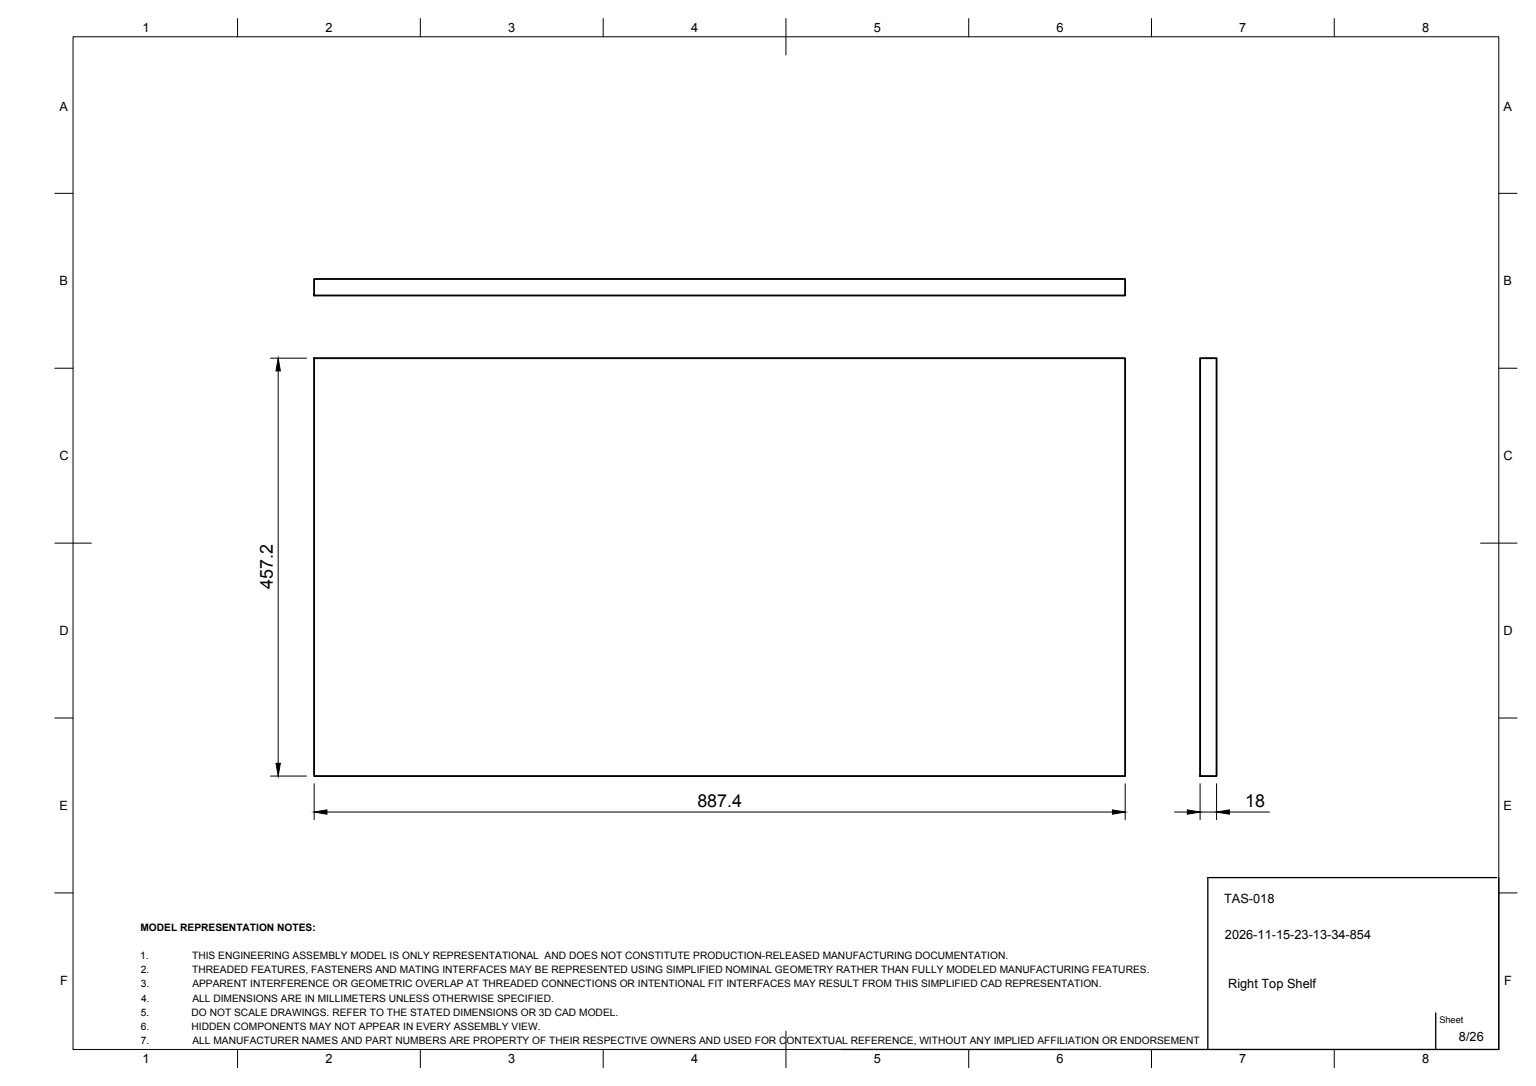
ISO-10303-21;
HEADER;
/* Generated by software containing ST-Developer
 * from STEP Tools, Inc. (www.steptools.com) 
 */

FILE_DESCRIPTION(
/* description */ (''),
/* implementation_level */ '2;1');

FILE_NAME(
/* name */ 'Right Top Shelf.step',
/* time_stamp */ '2026-11-15T15:17:57-08:00',
/* author */ (''),
/* organization */ (''),
/* preprocessor_version */ 'ST-DEVELOPER v20.2',
/* originating_system */ 'Autodesk Translation Framework v15.17.0.0',
/* authorisation */ '');

FILE_SCHEMA (('AUTOMOTIVE_DESIGN { 1 0 10303 214 3 1 1 }'));
ENDSEC;

DATA;
#10=MECHANICAL_DESIGN_GEOMETRIC_PRESENTATION_REPRESENTATION('',(#183),#3723);
#135=SHAPE_REPRESENTATION_RELATIONSHIP('SRR','None',#3816,#159);
#159=ADVANCED_BREP_SHAPE_REPRESENTATION('',(#207),#3705);
#183=STYLED_ITEM('',(#3947),#207);
#207=MANIFOLD_SOLID_BREP('Body1',#2031);
#258=FACE_OUTER_BOUND('',#384,.T.);
#259=FACE_OUTER_BOUND('',#385,.T.);
#260=FACE_OUTER_BOUND('',#386,.T.);
#261=FACE_OUTER_BOUND('',#387,.T.);
#262=FACE_OUTER_BOUND('',#388,.T.);
#263=FACE_OUTER_BOUND('',#389,.T.);
#384=EDGE_LOOP('',(#1437,#1438,#1439,#1440));
#385=EDGE_LOOP('',(#1441,#1442,#1443,#1444));
#386=EDGE_LOOP('',(#1445,#1446,#1447,#1448));
#387=EDGE_LOOP('',(#1449,#1450,#1451,#1452));
#388=EDGE_LOOP('',(#1453,#1454,#1455,#1456));
#389=EDGE_LOOP('',(#1457,#1458,#1459,#1460));
#538=LINE('',#3254,#760);
#539=LINE('',#3256,#761);
#540=LINE('',#3258,#762);
#541=LINE('',#3259,#763);
#542=LINE('',#3262,#764);
#543=LINE('',#3264,#765);
#544=LINE('',#3265,#766);
#545=LINE('',#3268,#767);
#546=LINE('',#3270,#768);
#547=LINE('',#3271,#769);
#548=LINE('',#3273,#770);
#549=LINE('',#3274,#771);
#760=VECTOR('',#2656,0.708661417322839);
#761=VECTOR('',#2657,18.);
#762=VECTOR('',#2658,0.708661417322839);
#763=VECTOR('',#2659,18.);
#764=VECTOR('',#2662,34.9370078740157);
#765=VECTOR('',#2663,18.);
#766=VECTOR('',#2664,34.9370078740157);
#767=VECTOR('',#2667,0.708661417322839);
#768=VECTOR('',#2668,18.);
#769=VECTOR('',#2669,0.708661417322839);
#770=VECTOR('',#2672,34.9370078740157);
#771=VECTOR('',#2673,34.9370078740157);
#963=VERTEX_POINT('',#3252);
#964=VERTEX_POINT('',#3253);
#965=VERTEX_POINT('',#3255);
#966=VERTEX_POINT('',#3257);
#967=VERTEX_POINT('',#3261);
#968=VERTEX_POINT('',#3263);
#969=VERTEX_POINT('',#3267);
#970=VERTEX_POINT('',#3269);
#1140=EDGE_CURVE('',#963,#964,#538,.T.);
#1141=EDGE_CURVE('',#965,#963,#539,.T.);
#1142=EDGE_CURVE('',#965,#966,#540,.T.);
#1143=EDGE_CURVE('',#966,#964,#541,.T.);
#1144=EDGE_CURVE('',#967,#963,#542,.T.);
#1145=EDGE_CURVE('',#968,#967,#543,.T.);
#1146=EDGE_CURVE('',#968,#965,#544,.T.);
#1147=EDGE_CURVE('',#967,#969,#545,.T.);
#1148=EDGE_CURVE('',#970,#969,#546,.T.);
#1149=EDGE_CURVE('',#968,#970,#547,.T.);
#1150=EDGE_CURVE('',#969,#964,#548,.T.);
#1151=EDGE_CURVE('',#970,#966,#549,.T.);
#1437=ORIENTED_EDGE('',*,*,#1140,.F.);
#1438=ORIENTED_EDGE('',*,*,#1141,.F.);
#1439=ORIENTED_EDGE('',*,*,#1142,.T.);
#1440=ORIENTED_EDGE('',*,*,#1143,.T.);
#1441=ORIENTED_EDGE('',*,*,#1144,.F.);
#1442=ORIENTED_EDGE('',*,*,#1145,.F.);
#1443=ORIENTED_EDGE('',*,*,#1146,.T.);
#1444=ORIENTED_EDGE('',*,*,#1141,.T.);
#1445=ORIENTED_EDGE('',*,*,#1147,.T.);
#1446=ORIENTED_EDGE('',*,*,#1148,.F.);
#1447=ORIENTED_EDGE('',*,*,#1149,.F.);
#1448=ORIENTED_EDGE('',*,*,#1145,.T.);
#1449=ORIENTED_EDGE('',*,*,#1150,.T.);
#1450=ORIENTED_EDGE('',*,*,#1143,.F.);
#1451=ORIENTED_EDGE('',*,*,#1151,.F.);
#1452=ORIENTED_EDGE('',*,*,#1148,.T.);
#1453=ORIENTED_EDGE('',*,*,#1142,.F.);
#1454=ORIENTED_EDGE('',*,*,#1146,.F.);
#1455=ORIENTED_EDGE('',*,*,#1149,.T.);
#1456=ORIENTED_EDGE('',*,*,#1151,.T.);
#1457=ORIENTED_EDGE('',*,*,#1140,.T.);
#1458=ORIENTED_EDGE('',*,*,#1150,.F.);
#1459=ORIENTED_EDGE('',*,*,#1147,.F.);
#1460=ORIENTED_EDGE('',*,*,#1144,.T.);
#1811=PLANE('',#2359);
#1812=PLANE('',#2360);
#1813=PLANE('',#2361);
#1814=PLANE('',#2362);
#1815=PLANE('',#2363);
#1816=PLANE('',#2364);
#1932=ADVANCED_FACE('',(#258),#1811,.T.);
#1933=ADVANCED_FACE('',(#259),#1812,.T.);
#1934=ADVANCED_FACE('',(#260),#1813,.F.);
#1935=ADVANCED_FACE('',(#261),#1814,.F.);
#1936=ADVANCED_FACE('',(#262),#1815,.T.);
#1937=ADVANCED_FACE('',(#263),#1816,.F.);
#2031=CLOSED_SHELL('',(#1932,#1933,#1934,#1935,#1936,#1937));
#2358=AXIS2_PLACEMENT_3D('',#3250,#2652,#2653);
#2359=AXIS2_PLACEMENT_3D('',#3251,#2654,#2655);
#2360=AXIS2_PLACEMENT_3D('',#3260,#2660,#2661);
#2361=AXIS2_PLACEMENT_3D('',#3266,#2665,#2666);
#2362=AXIS2_PLACEMENT_3D('',#3272,#2670,#2671);
#2363=AXIS2_PLACEMENT_3D('',#3275,#2674,#2675);
#2364=AXIS2_PLACEMENT_3D('',#3276,#2676,#2677);
#2652=DIRECTION('axis',(0.,0.,1.));
#2653=DIRECTION('refdir',(1.,0.,0.));
#2654=DIRECTION('center_axis',(1.,0.,0.));
#2655=DIRECTION('ref_axis',(0.,0.,-1.));
#2656=DIRECTION('',(0.,-1.,0.));
#2657=DIRECTION('',(0.,0.,-1.));
#2658=DIRECTION('',(0.,-1.,0.));
#2659=DIRECTION('',(0.,0.,-1.));
#2660=DIRECTION('center_axis',(0.,1.,0.));
#2661=DIRECTION('ref_axis',(0.,0.,1.));
#2662=DIRECTION('',(1.,0.,0.));
#2663=DIRECTION('',(0.,0.,-1.));
#2664=DIRECTION('',(1.,0.,0.));
#2665=DIRECTION('center_axis',(1.,0.,0.));
#2666=DIRECTION('ref_axis',(0.,0.,-1.));
#2667=DIRECTION('',(0.,-1.,0.));
#2668=DIRECTION('',(0.,0.,-1.));
#2669=DIRECTION('',(0.,-1.,0.));
#2670=DIRECTION('center_axis',(0.,1.,0.));
#2671=DIRECTION('ref_axis',(0.,0.,1.));
#2672=DIRECTION('',(1.,0.,0.));
#2673=DIRECTION('',(1.,0.,0.));
#2674=DIRECTION('center_axis',(0.,0.,1.));
#2675=DIRECTION('ref_axis',(1.,0.,0.));
#2676=DIRECTION('center_axis',(0.,0.,1.));
#2677=DIRECTION('ref_axis',(1.,0.,0.));
#3250=CARTESIAN_POINT('',(0.,0.,0.));
#3251=CARTESIAN_POINT('Origin',(35.2913385826772,0.,18.7086614173228));
#3252=CARTESIAN_POINT('',(35.2913385826772,67.3543307086614,0.708661417322834));
#3253=CARTESIAN_POINT('',(35.2913385826772,66.6456692913386,0.708661417322834));
#3254=CARTESIAN_POINT('',(35.2913385826772,67.3543307086614,0.708661417322834));
#3255=CARTESIAN_POINT('',(35.2913385826772,67.3543307086614,18.7086614173228));
#3256=CARTESIAN_POINT('',(35.2913385826772,67.3543307086614,18.7086614173228));
#3257=CARTESIAN_POINT('',(35.2913385826772,66.6456692913386,18.7086614173228));
#3258=CARTESIAN_POINT('',(35.2913385826772,67.3543307086614,18.7086614173228));
#3259=CARTESIAN_POINT('',(35.2913385826772,66.6456692913386,18.7086614173228));
#3260=CARTESIAN_POINT('Origin',(0.,67.3543307086614,18.7086614173228));
#3261=CARTESIAN_POINT('',(0.354330708661416,67.3543307086614,0.708661417322834));
#3262=CARTESIAN_POINT('',(0.354330708661416,67.3543307086614,0.708661417322834));
#3263=CARTESIAN_POINT('',(0.354330708661416,67.3543307086614,18.7086614173228));
#3264=CARTESIAN_POINT('',(0.354330708661416,67.3543307086614,18.7086614173228));
#3265=CARTESIAN_POINT('',(0.354330708661416,67.3543307086614,18.7086614173228));
#3266=CARTESIAN_POINT('Origin',(0.354330708661416,0.,18.7086614173228));
#3267=CARTESIAN_POINT('',(0.354330708661416,66.6456692913386,0.708661417322834));
#3268=CARTESIAN_POINT('',(0.354330708661416,67.3543307086614,0.708661417322834));
#3269=CARTESIAN_POINT('',(0.354330708661416,66.6456692913386,18.7086614173228));
#3270=CARTESIAN_POINT('',(0.354330708661416,66.6456692913386,18.7086614173228));
#3271=CARTESIAN_POINT('',(0.354330708661416,67.3543307086614,18.7086614173228));
#3272=CARTESIAN_POINT('Origin',(0.,66.6456692913386,18.7086614173228));
#3273=CARTESIAN_POINT('',(0.354330708661416,66.6456692913386,0.708661417322834));
#3274=CARTESIAN_POINT('',(0.354330708661416,66.6456692913386,18.7086614173228));
#3275=CARTESIAN_POINT('Origin',(0.,0.,18.7086614173228));
#3276=CARTESIAN_POINT('Origin',(0.,0.,0.708661417322834));
#3678=UNCERTAINTY_MEASURE_WITH_UNIT(LENGTH_MEASURE(0.000393700787401575),
#3725,'DISTANCE_ACCURACY_VALUE',
'Maximum model space distance between geometric entities at asserted c
onnectivities');
#3696=UNCERTAINTY_MEASURE_WITH_UNIT(LENGTH_MEASURE(0.000393700787401575),
#3725,'DISTANCE_ACCURACY_VALUE',
'Maximum model space distance between geometric entities at asserted c
onnectivities');
#3705=(
GEOMETRIC_REPRESENTATION_CONTEXT(3)
GLOBAL_UNCERTAINTY_ASSIGNED_CONTEXT((#3678))
GLOBAL_UNIT_ASSIGNED_CONTEXT((#3725,#3729,#3730))
REPRESENTATION_CONTEXT('','3D')
);
#3723=(
GEOMETRIC_REPRESENTATION_CONTEXT(3)
GLOBAL_UNCERTAINTY_ASSIGNED_CONTEXT((#3696))
GLOBAL_UNIT_ASSIGNED_CONTEXT((#3725,#3729,#3730))
REPRESENTATION_CONTEXT('','3D')
);
#3724=DIMENSIONAL_EXPONENTS(1.,0.,0.,0.,0.,0.,0.);
#3725=(
CONVERSION_BASED_UNIT('inch',#3728)
LENGTH_UNIT()
NAMED_UNIT(#3724)
);
#3726=(
LENGTH_UNIT()
NAMED_UNIT(*)
SI_UNIT(.MILLI.,.METRE.)
);
#3728=LENGTH_MEASURE_WITH_UNIT(LENGTH_MEASURE(25.4),#3726);
#3729=(
NAMED_UNIT(*)
PLANE_ANGLE_UNIT()
SI_UNIT($,.RADIAN.)
);
#3730=(
NAMED_UNIT(*)
SI_UNIT($,.STERADIAN.)
SOLID_ANGLE_UNIT()
);
#3739=SHAPE_DEFINITION_REPRESENTATION(#3766,#3816);
#3766=PRODUCT_DEFINITION_SHAPE('',$,#3843);
#3816=SHAPE_REPRESENTATION('',(#2358),#3705);
#3834=PRODUCT_DEFINITION_CONTEXT('part definition',#3914,'design');
#3843=PRODUCT_DEFINITION('2026-11-15-23-13-34-854','Right Top Shelf',#3869,
#3834);
#3869=PRODUCT_DEFINITION_FORMATION('',$,#3924);
#3914=APPLICATION_CONTEXT(
'Core Data for Automotive Mechanical Design Process');
#3915=PRODUCT_CONTEXT('part definition',#3914,'mechanical');
#3924=PRODUCT('2026-11-15-23-13-34-854','Right Top Shelf',$,(#3915));
#3947=PRESENTATION_STYLE_ASSIGNMENT((#3955));
#3955=SURFACE_STYLE_USAGE(.BOTH.,#3963);
#3963=SURFACE_SIDE_STYLE('',(#3971));
#3971=SURFACE_STYLE_FILL_AREA(#3979);
#3979=FILL_AREA_STYLE('Light Blue',(#3987));
#3987=FILL_AREA_STYLE_COLOUR('Light Blue',#3995);
#3995=COLOUR_RGB('Light Blue',0.67843137254902,0.847058823529412,0.901960784313726);
ENDSEC;
END-ISO-10303-21;
